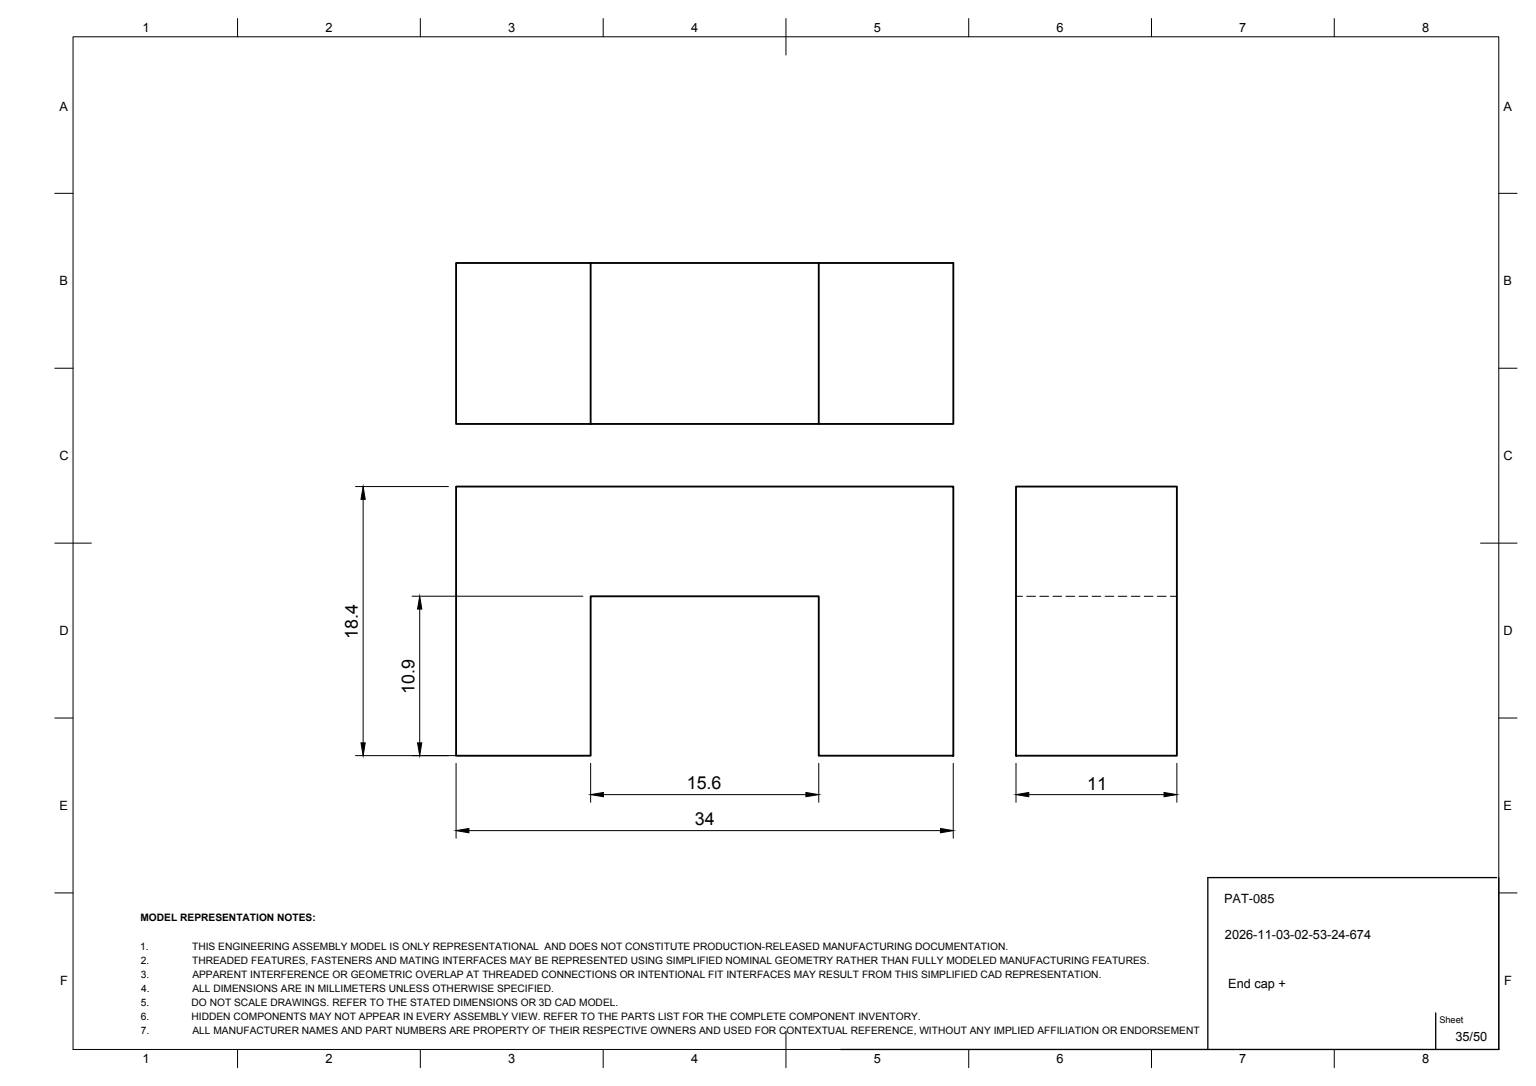
ISO-10303-21;
HEADER;
/* Generated by software containing ST-Developer
 * from STEP Tools, Inc. (www.steptools.com) 
 */

FILE_DESCRIPTION(
/* description */ ('Rack and pinion manual slide'),
/* implementation_level */ '2;1');

FILE_NAME(
/* name */ 'End cap +.step',
/* time_stamp */ '2026-10-28T03:22:49-07:00',
/* author */ (''),
/* organization */ (''),
/* preprocessor_version */ 'ST-DEVELOPER v20.2',
/* originating_system */ 'Autodesk Translation Framework v15.17.0.0',
/* authorisation */ '');

FILE_SCHEMA (('AUTOMOTIVE_DESIGN { 1 0 10303 214 3 1 1 }'));
ENDSEC;

DATA;
#10=MECHANICAL_DESIGN_GEOMETRIC_PRESENTATION_REPRESENTATION('',(#767),#34851);
#668=SHAPE_REPRESENTATION_RELATIONSHIP('SRR','None',#35106,#714);
#714=ADVANCED_BREP_SHAPE_REPRESENTATION('',(#818),#34831);
#767=STYLED_ITEM('',(#35404),#818);
#818=MANIFOLD_SOLID_BREP('Body1',#13789);
#1403=PLANE('',#15150);
#1404=PLANE('',#15151);
#1405=PLANE('',#15152);
#1406=PLANE('',#15153);
#1407=PLANE('',#15154);
#1408=PLANE('',#15155);
#1409=PLANE('',#15156);
#1410=PLANE('',#15157);
#1411=PLANE('',#15158);
#1412=PLANE('',#15159);
#2036=FACE_OUTER_BOUND('',#2951,.T.);
#2037=FACE_OUTER_BOUND('',#2952,.T.);
#2038=FACE_OUTER_BOUND('',#2953,.T.);
#2039=FACE_OUTER_BOUND('',#2954,.T.);
#2040=FACE_OUTER_BOUND('',#2955,.T.);
#2041=FACE_OUTER_BOUND('',#2956,.T.);
#2042=FACE_OUTER_BOUND('',#2957,.T.);
#2043=FACE_OUTER_BOUND('',#2958,.T.);
#2044=FACE_OUTER_BOUND('',#2959,.T.);
#2045=FACE_OUTER_BOUND('',#2960,.T.);
#2951=EDGE_LOOP('',(#11756,#11757,#11758,#11759));
#2952=EDGE_LOOP('',(#11760,#11761,#11762,#11763));
#2953=EDGE_LOOP('',(#11764,#11765,#11766,#11767));
#2954=EDGE_LOOP('',(#11768,#11769,#11770,#11771));
#2955=EDGE_LOOP('',(#11772,#11773,#11774,#11775));
#2956=EDGE_LOOP('',(#11776,#11777,#11778,#11779));
#2957=EDGE_LOOP('',(#11780,#11781,#11782,#11783));
#2958=EDGE_LOOP('',(#11784,#11785,#11786,#11787));
#2959=EDGE_LOOP('',(#11788,#11789,#11790,#11791,#11792,#11793,#11794,#11795));
#2960=EDGE_LOOP('',(#11796,#11797,#11798,#11799,#11800,#11801,#11802,#11803));
#4178=LINE('',#22401,#5469);
#4179=LINE('',#22403,#5470);
#4180=LINE('',#22405,#5471);
#4181=LINE('',#22406,#5472);
#4182=LINE('',#22409,#5473);
#4183=LINE('',#22411,#5474);
#4184=LINE('',#22412,#5475);
#4185=LINE('',#22415,#5476);
#4186=LINE('',#22417,#5477);
#4187=LINE('',#22418,#5478);
#4188=LINE('',#22421,#5479);
#4189=LINE('',#22423,#5480);
#4190=LINE('',#22424,#5481);
#4191=LINE('',#22427,#5482);
#4192=LINE('',#22429,#5483);
#4193=LINE('',#22430,#5484);
#4194=LINE('',#22433,#5485);
#4195=LINE('',#22435,#5486);
#4196=LINE('',#22436,#5487);
#4197=LINE('',#22439,#5488);
#4198=LINE('',#22441,#5489);
#4199=LINE('',#22442,#5490);
#4200=LINE('',#22444,#5491);
#4201=LINE('',#22445,#5492);
#5469=VECTOR('',#18222,1.);
#5470=VECTOR('',#18223,1.);
#5471=VECTOR('',#18224,1.);
#5472=VECTOR('',#18225,1.);
#5473=VECTOR('',#18228,1.);
#5474=VECTOR('',#18229,1.);
#5475=VECTOR('',#18230,1.);
#5476=VECTOR('',#18233,1.);
#5477=VECTOR('',#18234,1.);
#5478=VECTOR('',#18235,1.);
#5479=VECTOR('',#18238,1.);
#5480=VECTOR('',#18239,1.);
#5481=VECTOR('',#18240,1.);
#5482=VECTOR('',#18243,1.);
#5483=VECTOR('',#18244,1.);
#5484=VECTOR('',#18245,1.);
#5485=VECTOR('',#18248,1.);
#5486=VECTOR('',#18249,1.);
#5487=VECTOR('',#18250,1.);
#5488=VECTOR('',#18253,1.);
#5489=VECTOR('',#18254,1.);
#5490=VECTOR('',#18255,1.);
#5491=VECTOR('',#18258,1.);
#5492=VECTOR('',#18259,1.);
#7070=VERTEX_POINT('',#22399);
#7071=VERTEX_POINT('',#22400);
#7072=VERTEX_POINT('',#22402);
#7073=VERTEX_POINT('',#22404);
#7074=VERTEX_POINT('',#22408);
#7075=VERTEX_POINT('',#22410);
#7076=VERTEX_POINT('',#22414);
#7077=VERTEX_POINT('',#22416);
#7078=VERTEX_POINT('',#22420);
#7079=VERTEX_POINT('',#22422);
#7080=VERTEX_POINT('',#22426);
#7081=VERTEX_POINT('',#22428);
#7082=VERTEX_POINT('',#22432);
#7083=VERTEX_POINT('',#22434);
#7084=VERTEX_POINT('',#22438);
#7085=VERTEX_POINT('',#22440);
#8690=EDGE_CURVE('',#7070,#7071,#4178,.T.);
#8691=EDGE_CURVE('',#7071,#7072,#4179,.T.);
#8692=EDGE_CURVE('',#7073,#7072,#4180,.T.);
#8693=EDGE_CURVE('',#7070,#7073,#4181,.T.);
#8694=EDGE_CURVE('',#7074,#7070,#4182,.T.);
#8695=EDGE_CURVE('',#7075,#7073,#4183,.T.);
#8696=EDGE_CURVE('',#7074,#7075,#4184,.T.);
#8697=EDGE_CURVE('',#7076,#7074,#4185,.T.);
#8698=EDGE_CURVE('',#7077,#7075,#4186,.T.);
#8699=EDGE_CURVE('',#7076,#7077,#4187,.T.);
#8700=EDGE_CURVE('',#7078,#7076,#4188,.T.);
#8701=EDGE_CURVE('',#7079,#7077,#4189,.T.);
#8702=EDGE_CURVE('',#7078,#7079,#4190,.T.);
#8703=EDGE_CURVE('',#7080,#7078,#4191,.T.);
#8704=EDGE_CURVE('',#7081,#7079,#4192,.T.);
#8705=EDGE_CURVE('',#7080,#7081,#4193,.T.);
#8706=EDGE_CURVE('',#7082,#7080,#4194,.T.);
#8707=EDGE_CURVE('',#7083,#7081,#4195,.T.);
#8708=EDGE_CURVE('',#7082,#7083,#4196,.T.);
#8709=EDGE_CURVE('',#7084,#7082,#4197,.T.);
#8710=EDGE_CURVE('',#7085,#7083,#4198,.T.);
#8711=EDGE_CURVE('',#7084,#7085,#4199,.T.);
#8712=EDGE_CURVE('',#7071,#7084,#4200,.T.);
#8713=EDGE_CURVE('',#7072,#7085,#4201,.T.);
#11756=ORIENTED_EDGE('',*,*,#8690,.T.);
#11757=ORIENTED_EDGE('',*,*,#8691,.T.);
#11758=ORIENTED_EDGE('',*,*,#8692,.F.);
#11759=ORIENTED_EDGE('',*,*,#8693,.F.);
#11760=ORIENTED_EDGE('',*,*,#8694,.T.);
#11761=ORIENTED_EDGE('',*,*,#8693,.T.);
#11762=ORIENTED_EDGE('',*,*,#8695,.F.);
#11763=ORIENTED_EDGE('',*,*,#8696,.F.);
#11764=ORIENTED_EDGE('',*,*,#8697,.T.);
#11765=ORIENTED_EDGE('',*,*,#8696,.T.);
#11766=ORIENTED_EDGE('',*,*,#8698,.F.);
#11767=ORIENTED_EDGE('',*,*,#8699,.F.);
#11768=ORIENTED_EDGE('',*,*,#8700,.T.);
#11769=ORIENTED_EDGE('',*,*,#8699,.T.);
#11770=ORIENTED_EDGE('',*,*,#8701,.F.);
#11771=ORIENTED_EDGE('',*,*,#8702,.F.);
#11772=ORIENTED_EDGE('',*,*,#8703,.T.);
#11773=ORIENTED_EDGE('',*,*,#8702,.T.);
#11774=ORIENTED_EDGE('',*,*,#8704,.F.);
#11775=ORIENTED_EDGE('',*,*,#8705,.F.);
#11776=ORIENTED_EDGE('',*,*,#8706,.T.);
#11777=ORIENTED_EDGE('',*,*,#8705,.T.);
#11778=ORIENTED_EDGE('',*,*,#8707,.F.);
#11779=ORIENTED_EDGE('',*,*,#8708,.F.);
#11780=ORIENTED_EDGE('',*,*,#8709,.T.);
#11781=ORIENTED_EDGE('',*,*,#8708,.T.);
#11782=ORIENTED_EDGE('',*,*,#8710,.F.);
#11783=ORIENTED_EDGE('',*,*,#8711,.F.);
#11784=ORIENTED_EDGE('',*,*,#8712,.T.);
#11785=ORIENTED_EDGE('',*,*,#8711,.T.);
#11786=ORIENTED_EDGE('',*,*,#8713,.F.);
#11787=ORIENTED_EDGE('',*,*,#8691,.F.);
#11788=ORIENTED_EDGE('',*,*,#8713,.T.);
#11789=ORIENTED_EDGE('',*,*,#8710,.T.);
#11790=ORIENTED_EDGE('',*,*,#8707,.T.);
#11791=ORIENTED_EDGE('',*,*,#8704,.T.);
#11792=ORIENTED_EDGE('',*,*,#8701,.T.);
#11793=ORIENTED_EDGE('',*,*,#8698,.T.);
#11794=ORIENTED_EDGE('',*,*,#8695,.T.);
#11795=ORIENTED_EDGE('',*,*,#8692,.T.);
#11796=ORIENTED_EDGE('',*,*,#8712,.F.);
#11797=ORIENTED_EDGE('',*,*,#8690,.F.);
#11798=ORIENTED_EDGE('',*,*,#8694,.F.);
#11799=ORIENTED_EDGE('',*,*,#8697,.F.);
#11800=ORIENTED_EDGE('',*,*,#8700,.F.);
#11801=ORIENTED_EDGE('',*,*,#8703,.F.);
#11802=ORIENTED_EDGE('',*,*,#8706,.F.);
#11803=ORIENTED_EDGE('',*,*,#8709,.F.);
#13514=ADVANCED_FACE('',(#2036),#1403,.T.);
#13515=ADVANCED_FACE('',(#2037),#1404,.T.);
#13516=ADVANCED_FACE('',(#2038),#1405,.T.);
#13517=ADVANCED_FACE('',(#2039),#1406,.T.);
#13518=ADVANCED_FACE('',(#2040),#1407,.T.);
#13519=ADVANCED_FACE('',(#2041),#1408,.T.);
#13520=ADVANCED_FACE('',(#2042),#1409,.T.);
#13521=ADVANCED_FACE('',(#2043),#1410,.T.);
#13522=ADVANCED_FACE('',(#2044),#1411,.T.);
#13523=ADVANCED_FACE('',(#2045),#1412,.F.);
#13789=CLOSED_SHELL('',(#13514,#13515,#13516,#13517,#13518,#13519,#13520,
#13521,#13522,#13523));
#15149=AXIS2_PLACEMENT_3D('',#22397,#18218,#18219);
#15150=AXIS2_PLACEMENT_3D('',#22398,#18220,#18221);
#15151=AXIS2_PLACEMENT_3D('',#22407,#18226,#18227);
#15152=AXIS2_PLACEMENT_3D('',#22413,#18231,#18232);
#15153=AXIS2_PLACEMENT_3D('',#22419,#18236,#18237);
#15154=AXIS2_PLACEMENT_3D('',#22425,#18241,#18242);
#15155=AXIS2_PLACEMENT_3D('',#22431,#18246,#18247);
#15156=AXIS2_PLACEMENT_3D('',#22437,#18251,#18252);
#15157=AXIS2_PLACEMENT_3D('',#22443,#18256,#18257);
#15158=AXIS2_PLACEMENT_3D('',#22446,#18260,#18261);
#15159=AXIS2_PLACEMENT_3D('',#22447,#18262,#18263);
#18218=DIRECTION('axis',(0.,0.,1.));
#18219=DIRECTION('refdir',(1.,0.,0.));
#18220=DIRECTION('center_axis',(0.,0.,1.));
#18221=DIRECTION('ref_axis',(0.,-1.,0.));
#18222=DIRECTION('',(0.,-1.,0.));
#18223=DIRECTION('',(1.,0.,0.));
#18224=DIRECTION('',(0.,-1.,0.));
#18225=DIRECTION('',(1.,0.,0.));
#18226=DIRECTION('center_axis',(0.,1.,0.));
#18227=DIRECTION('ref_axis',(0.,0.,1.));
#18228=DIRECTION('',(0.,0.,1.));
#18229=DIRECTION('',(0.,0.,1.));
#18230=DIRECTION('',(1.,0.,0.));
#18231=DIRECTION('center_axis',(0.,0.,-1.));
#18232=DIRECTION('ref_axis',(0.,1.,0.));
#18233=DIRECTION('',(0.,1.,0.));
#18234=DIRECTION('',(0.,1.,0.));
#18235=DIRECTION('',(1.,0.,0.));
#18236=DIRECTION('center_axis',(0.,-1.,0.));
#18237=DIRECTION('ref_axis',(0.,0.,-1.));
#18238=DIRECTION('',(0.,0.,-1.));
#18239=DIRECTION('',(0.,0.,-1.));
#18240=DIRECTION('',(1.,0.,0.));
#18241=DIRECTION('center_axis',(0.,0.,-1.));
#18242=DIRECTION('ref_axis',(0.,1.,0.));
#18243=DIRECTION('',(0.,1.,0.));
#18244=DIRECTION('',(0.,1.,0.));
#18245=DIRECTION('',(1.,0.,0.));
#18246=DIRECTION('center_axis',(0.,1.,0.));
#18247=DIRECTION('ref_axis',(0.,0.,1.));
#18248=DIRECTION('',(0.,0.,1.));
#18249=DIRECTION('',(0.,0.,1.));
#18250=DIRECTION('',(1.,0.,0.));
#18251=DIRECTION('center_axis',(0.,0.,-1.));
#18252=DIRECTION('ref_axis',(0.,1.,0.));
#18253=DIRECTION('',(0.,1.,0.));
#18254=DIRECTION('',(0.,1.,0.));
#18255=DIRECTION('',(1.,0.,0.));
#18256=DIRECTION('center_axis',(0.,-1.,0.));
#18257=DIRECTION('ref_axis',(0.,0.,-1.));
#18258=DIRECTION('',(0.,0.,-1.));
#18259=DIRECTION('',(0.,0.,-1.));
#18260=DIRECTION('center_axis',(1.,0.,0.));
#18261=DIRECTION('ref_axis',(0.,0.,-1.));
#18262=DIRECTION('center_axis',(1.,0.,0.));
#18263=DIRECTION('ref_axis',(0.,0.,-1.));
#22397=CARTESIAN_POINT('',(0.,0.,0.));
#22398=CARTESIAN_POINT('Origin',(1.97,1.7,2.3));
#22399=CARTESIAN_POINT('',(1.97,1.7,2.3));
#22400=CARTESIAN_POINT('',(1.97,-1.7,2.3));
#22401=CARTESIAN_POINT('',(1.97,1.7,2.3));
#22402=CARTESIAN_POINT('',(3.07,-1.7,2.3));
#22403=CARTESIAN_POINT('',(1.97,-1.7,2.3));
#22404=CARTESIAN_POINT('',(3.07,1.7,2.3));
#22405=CARTESIAN_POINT('',(3.07,1.7,2.3));
#22406=CARTESIAN_POINT('',(1.97,1.7,2.3));
#22407=CARTESIAN_POINT('Origin',(1.97,1.7,0.46));
#22408=CARTESIAN_POINT('',(1.97,1.7,0.46));
#22409=CARTESIAN_POINT('',(1.97,1.7,0.46));
#22410=CARTESIAN_POINT('',(3.07,1.7,0.46));
#22411=CARTESIAN_POINT('',(3.07,1.7,0.46));
#22412=CARTESIAN_POINT('',(1.97,1.7,0.46));
#22413=CARTESIAN_POINT('Origin',(1.97,0.78,0.46));
#22414=CARTESIAN_POINT('',(1.97,0.78,0.46));
#22415=CARTESIAN_POINT('',(1.97,0.78,0.46));
#22416=CARTESIAN_POINT('',(3.07,0.78,0.46));
#22417=CARTESIAN_POINT('',(3.07,0.78,0.46));
#22418=CARTESIAN_POINT('',(1.97,0.78,0.46));
#22419=CARTESIAN_POINT('Origin',(1.97,0.78,1.55));
#22420=CARTESIAN_POINT('',(1.97,0.78,1.55));
#22421=CARTESIAN_POINT('',(1.97,0.78,1.55));
#22422=CARTESIAN_POINT('',(3.07,0.78,1.55));
#22423=CARTESIAN_POINT('',(3.07,0.78,1.55));
#22424=CARTESIAN_POINT('',(1.97,0.78,1.55));
#22425=CARTESIAN_POINT('Origin',(1.97,-0.78,1.55));
#22426=CARTESIAN_POINT('',(1.97,-0.78,1.55));
#22427=CARTESIAN_POINT('',(1.97,-0.78,1.55));
#22428=CARTESIAN_POINT('',(3.07,-0.78,1.55));
#22429=CARTESIAN_POINT('',(3.07,-0.78,1.55));
#22430=CARTESIAN_POINT('',(1.97,-0.78,1.55));
#22431=CARTESIAN_POINT('Origin',(1.97,-0.78,0.46));
#22432=CARTESIAN_POINT('',(1.97,-0.78,0.46));
#22433=CARTESIAN_POINT('',(1.97,-0.78,0.46));
#22434=CARTESIAN_POINT('',(3.07,-0.78,0.46));
#22435=CARTESIAN_POINT('',(3.07,-0.78,0.46));
#22436=CARTESIAN_POINT('',(1.97,-0.78,0.46));
#22437=CARTESIAN_POINT('Origin',(1.97,-1.7,0.46));
#22438=CARTESIAN_POINT('',(1.97,-1.7,0.46));
#22439=CARTESIAN_POINT('',(1.97,-1.7,0.46));
#22440=CARTESIAN_POINT('',(3.07,-1.7,0.46));
#22441=CARTESIAN_POINT('',(3.07,-1.7,0.46));
#22442=CARTESIAN_POINT('',(1.97,-1.7,0.46));
#22443=CARTESIAN_POINT('Origin',(1.97,-1.7,2.3));
#22444=CARTESIAN_POINT('',(1.97,-1.7,2.3));
#22445=CARTESIAN_POINT('',(3.07,-1.7,2.3));
#22446=CARTESIAN_POINT('Origin',(3.07,0.,1.38));
#22447=CARTESIAN_POINT('Origin',(1.97,0.,1.38));
#34777=UNCERTAINTY_MEASURE_WITH_UNIT(LENGTH_MEASURE(0.001),#34852,
'DISTANCE_ACCURACY_VALUE',
'Maximum model space distance between geometric entities at asserted c
onnectivities');
#34797=UNCERTAINTY_MEASURE_WITH_UNIT(LENGTH_MEASURE(0.001),#34852,
'DISTANCE_ACCURACY_VALUE',
'Maximum model space distance between geometric entities at asserted c
onnectivities');
#34831=(
GEOMETRIC_REPRESENTATION_CONTEXT(3)
GLOBAL_UNCERTAINTY_ASSIGNED_CONTEXT((#34777))
GLOBAL_UNIT_ASSIGNED_CONTEXT((#34852,#34854,#34855))
REPRESENTATION_CONTEXT('','3D')
);
#34851=(
GEOMETRIC_REPRESENTATION_CONTEXT(3)
GLOBAL_UNCERTAINTY_ASSIGNED_CONTEXT((#34797))
GLOBAL_UNIT_ASSIGNED_CONTEXT((#34852,#34854,#34855))
REPRESENTATION_CONTEXT('','3D')
);
#34852=(
LENGTH_UNIT()
NAMED_UNIT(*)
SI_UNIT(.CENTI.,.METRE.)
);
#34854=(
NAMED_UNIT(*)
PLANE_ANGLE_UNIT()
SI_UNIT($,.RADIAN.)
);
#34855=(
NAMED_UNIT(*)
SI_UNIT($,.STERADIAN.)
SOLID_ANGLE_UNIT()
);
#34889=SHAPE_DEFINITION_REPRESENTATION(#34947,#35106);
#34947=PRODUCT_DEFINITION_SHAPE('',$,#35160);
#35106=SHAPE_REPRESENTATION('',(#15149),#34831);
#35126=PRODUCT_DEFINITION_CONTEXT('part definition',#35287,'design');
#35160=PRODUCT_DEFINITION('End cap +','End cap +',#35213,#35126);
#35213=PRODUCT_DEFINITION_FORMATION('',$,#35322);
#35287=APPLICATION_CONTEXT(
'Core Data for Automotive Mechanical Design Process');
#35288=PRODUCT_CONTEXT('part definition',#35287,'mechanical');
#35322=PRODUCT('End cap +','End cap +','End cap +',(#35288));
#35398=COLOUR_RGB('Sky Blue',0.24,0.69,0.87);
#35399=FILL_AREA_STYLE_COLOUR('',#35398);
#35400=FILL_AREA_STYLE('',(#35399));
#35401=SURFACE_STYLE_FILL_AREA(#35400);
#35402=SURFACE_SIDE_STYLE('',(#35401));
#35403=SURFACE_STYLE_USAGE(.BOTH.,#35402);
#35404=PRESENTATION_STYLE_ASSIGNMENT((#35403));
ENDSEC;
END-ISO-10303-21;
